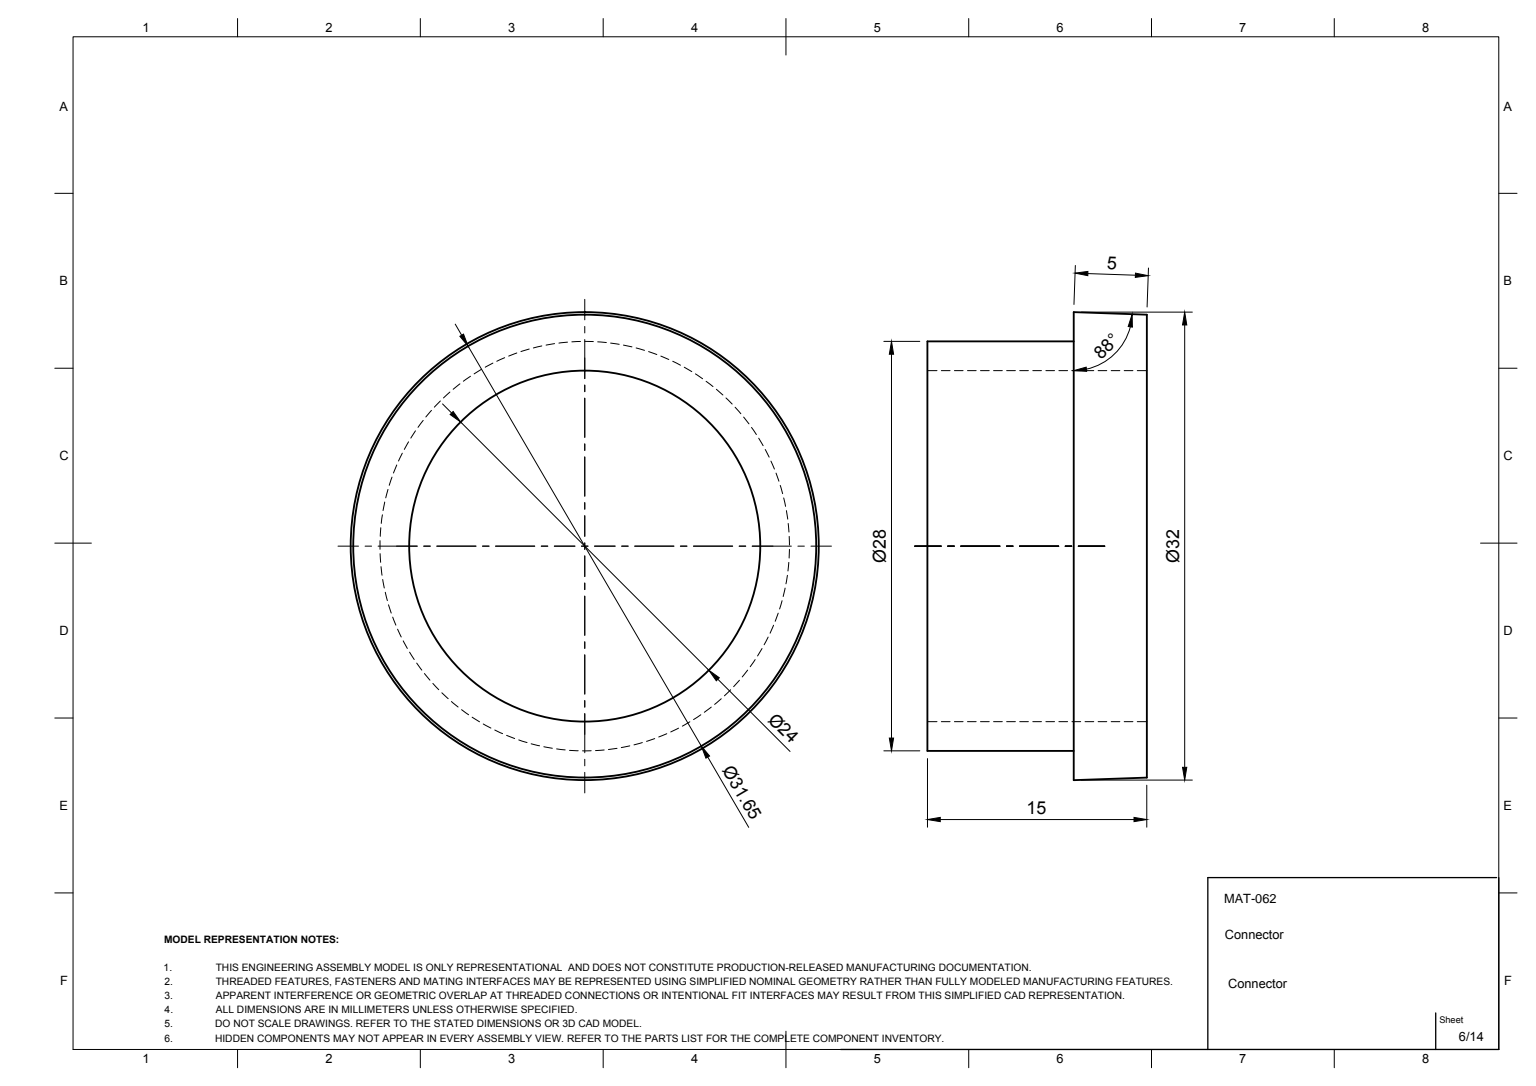
ISO-10303-21;
HEADER;
/* Generated by software containing ST-Developer
 * from STEP Tools, Inc. (www.steptools.com) 
 */

FILE_DESCRIPTION(
/* description */ (''),
/* implementation_level */ '2;1');

FILE_NAME(
/* name */ 'Connector.step',
/* time_stamp */ '2026-10-24T10:18:25-07:00',
/* author */ (''),
/* organization */ (''),
/* preprocessor_version */ 'ST-DEVELOPER v20.2',
/* originating_system */ 'Autodesk Translation Framework v15.15.0.0',
/* authorisation */ '');

FILE_SCHEMA (('AUTOMOTIVE_DESIGN { 1 0 10303 214 3 1 1 }'));
ENDSEC;

DATA;
#10=MECHANICAL_DESIGN_GEOMETRIC_PRESENTATION_REPRESENTATION('',(#265),#14125);
#198=CONICAL_SURFACE('',#6890,16.,0.0349065850398866);
#236=SHAPE_REPRESENTATION_RELATIONSHIP('SRR','None',#14210,#246);
#246=ADVANCED_BREP_SHAPE_REPRESENTATION('',(#278),#14124);
#265=STYLED_ITEM('',(#14263),#278);
#278=MANIFOLD_SOLID_BREP('Connector',#6146);
#625=CYLINDRICAL_SURFACE('',#6897,14.);
#626=CYLINDRICAL_SURFACE('',#6901,12.);
#729=FACE_BOUND('',#1536,.T.);
#730=FACE_BOUND('',#1538,.T.);
#731=FACE_BOUND('',#1541,.T.);
#1079=FACE_OUTER_BOUND('',#1534,.T.);
#1080=FACE_OUTER_BOUND('',#1535,.T.);
#1081=FACE_OUTER_BOUND('',#1537,.T.);
#1082=FACE_OUTER_BOUND('',#1539,.T.);
#1083=FACE_OUTER_BOUND('',#1540,.T.);
#1084=FACE_OUTER_BOUND('',#1542,.T.);
#1534=EDGE_LOOP('',(#5609,#5610,#5611,#5612));
#1535=EDGE_LOOP('',(#5613));
#1536=EDGE_LOOP('',(#5614));
#1537=EDGE_LOOP('',(#5615));
#1538=EDGE_LOOP('',(#5616));
#1539=EDGE_LOOP('',(#5617,#5618,#5619,#5620));
#1540=EDGE_LOOP('',(#5621));
#1541=EDGE_LOOP('',(#5622));
#1542=EDGE_LOOP('',(#5623,#5624,#5625,#5626));
#1797=CIRCLE('',#6891,16.);
#1798=CIRCLE('',#6892,15.8253961525413);
#1799=CIRCLE('',#6894,12.);
#1800=CIRCLE('',#6896,14.);
#1801=CIRCLE('',#6898,14.);
#1802=CIRCLE('',#6900,12.);
#2188=LINE('',#14078,#2576);
#2189=LINE('',#14088,#2577);
#2190=LINE('',#14094,#2578);
#2576=VECTOR('',#8560,16.);
#2577=VECTOR('',#8573,14.);
#2578=VECTOR('',#8582,12.);
#3122=VERTEX_POINT('',#14075);
#3123=VERTEX_POINT('',#14077);
#3124=VERTEX_POINT('',#14081);
#3125=VERTEX_POINT('',#14084);
#3126=VERTEX_POINT('',#14087);
#3127=VERTEX_POINT('',#14091);
#3952=EDGE_CURVE('',#3122,#3122,#1797,.T.);
#3953=EDGE_CURVE('',#3122,#3123,#2188,.T.);
#3954=EDGE_CURVE('',#3123,#3123,#1798,.T.);
#3955=EDGE_CURVE('',#3124,#3124,#1799,.T.);
#3956=EDGE_CURVE('',#3125,#3125,#1800,.T.);
#3957=EDGE_CURVE('',#3125,#3126,#2189,.T.);
#3958=EDGE_CURVE('',#3126,#3126,#1801,.T.);
#3959=EDGE_CURVE('',#3127,#3127,#1802,.T.);
#3960=EDGE_CURVE('',#3124,#3127,#2190,.T.);
#5609=ORIENTED_EDGE('',*,*,#3952,.F.);
#5610=ORIENTED_EDGE('',*,*,#3953,.T.);
#5611=ORIENTED_EDGE('',*,*,#3954,.T.);
#5612=ORIENTED_EDGE('',*,*,#3953,.F.);
#5613=ORIENTED_EDGE('',*,*,#3954,.F.);
#5614=ORIENTED_EDGE('',*,*,#3955,.T.);
#5615=ORIENTED_EDGE('',*,*,#3952,.T.);
#5616=ORIENTED_EDGE('',*,*,#3956,.F.);
#5617=ORIENTED_EDGE('',*,*,#3956,.T.);
#5618=ORIENTED_EDGE('',*,*,#3957,.T.);
#5619=ORIENTED_EDGE('',*,*,#3958,.F.);
#5620=ORIENTED_EDGE('',*,*,#3957,.F.);
#5621=ORIENTED_EDGE('',*,*,#3958,.T.);
#5622=ORIENTED_EDGE('',*,*,#3959,.F.);
#5623=ORIENTED_EDGE('',*,*,#3955,.F.);
#5624=ORIENTED_EDGE('',*,*,#3960,.T.);
#5625=ORIENTED_EDGE('',*,*,#3959,.T.);
#5626=ORIENTED_EDGE('',*,*,#3960,.F.);
#5778=PLANE('',#6893);
#5779=PLANE('',#6895);
#5780=PLANE('',#6899);
#6128=ADVANCED_FACE('',(#1079),#198,.T.);
#6129=ADVANCED_FACE('',(#1080,#729),#5778,.F.);
#6130=ADVANCED_FACE('',(#1081,#730),#5779,.T.);
#6131=ADVANCED_FACE('',(#1082),#625,.T.);
#6132=ADVANCED_FACE('',(#1083,#731),#5780,.T.);
#6133=ADVANCED_FACE('',(#1084),#626,.F.);
#6146=CLOSED_SHELL('',(#6128,#6129,#6130,#6131,#6132,#6133));
#6889=AXIS2_PLACEMENT_3D('',#14073,#8554,#8555);
#6890=AXIS2_PLACEMENT_3D('',#14074,#8556,#8557);
#6891=AXIS2_PLACEMENT_3D('',#14076,#8558,#8559);
#6892=AXIS2_PLACEMENT_3D('',#14079,#8561,#8562);
#6893=AXIS2_PLACEMENT_3D('',#14080,#8563,#8564);
#6894=AXIS2_PLACEMENT_3D('',#14082,#8565,#8566);
#6895=AXIS2_PLACEMENT_3D('',#14083,#8567,#8568);
#6896=AXIS2_PLACEMENT_3D('',#14085,#8569,#8570);
#6897=AXIS2_PLACEMENT_3D('',#14086,#8571,#8572);
#6898=AXIS2_PLACEMENT_3D('',#14089,#8574,#8575);
#6899=AXIS2_PLACEMENT_3D('',#14090,#8576,#8577);
#6900=AXIS2_PLACEMENT_3D('',#14092,#8578,#8579);
#6901=AXIS2_PLACEMENT_3D('',#14093,#8580,#8581);
#8554=DIRECTION('axis',(0.,0.,1.));
#8555=DIRECTION('refdir',(1.,0.,0.));
#8556=DIRECTION('center_axis',(0.,-1.,0.));
#8557=DIRECTION('ref_axis',(0.,0.,-1.));
#8558=DIRECTION('center_axis',(0.,-1.,0.));
#8559=DIRECTION('ref_axis',(0.,0.,-1.));
#8560=DIRECTION('',(4.27395569285715E-18,0.999390827019096,-0.034899496702501));
#8561=DIRECTION('center_axis',(0.,-1.,0.));
#8562=DIRECTION('ref_axis',(0.,0.,-1.));
#8563=DIRECTION('center_axis',(0.,-1.,0.));
#8564=DIRECTION('ref_axis',(0.,0.,-1.));
#8565=DIRECTION('center_axis',(0.,-1.,0.));
#8566=DIRECTION('ref_axis',(0.,0.,-1.));
#8567=DIRECTION('center_axis',(0.,-1.,0.));
#8568=DIRECTION('ref_axis',(0.,0.,-1.));
#8569=DIRECTION('center_axis',(0.,-1.,0.));
#8570=DIRECTION('ref_axis',(0.,0.,-1.));
#8571=DIRECTION('center_axis',(0.,1.,0.));
#8572=DIRECTION('ref_axis',(0.,0.,1.));
#8573=DIRECTION('',(0.,-1.,0.));
#8574=DIRECTION('center_axis',(0.,-1.,0.));
#8575=DIRECTION('ref_axis',(0.,0.,-1.));
#8576=DIRECTION('center_axis',(0.,-1.,0.));
#8577=DIRECTION('ref_axis',(0.,0.,-1.));
#8578=DIRECTION('center_axis',(0.,-1.,0.));
#8579=DIRECTION('ref_axis',(0.,0.,-1.));
#8580=DIRECTION('center_axis',(0.,-1.,0.));
#8581=DIRECTION('ref_axis',(0.,0.,-1.));
#8582=DIRECTION('',(0.,-1.,0.));
#14073=CARTESIAN_POINT('',(0.,0.,0.));
#14074=CARTESIAN_POINT('Origin',(0.,89.,-11.9999999999999));
#14075=CARTESIAN_POINT('',(-1.95943487863577E-15,89.,4.00000000000008));
#14076=CARTESIAN_POINT('Origin',(0.,89.,-11.9999999999999));
#14077=CARTESIAN_POINT('',(-1.93805207434485E-15,94.,3.82539615254134));
#14078=CARTESIAN_POINT('',(-1.95943487863577E-15,89.,4.00000000000008));
#14079=CARTESIAN_POINT('Origin',(0.,94.,-11.9999999999999));
#14080=CARTESIAN_POINT('Origin',(0.,94.,-11.9999999999999));
#14081=CARTESIAN_POINT('',(-1.46957615897682E-15,94.,8.21565038222616E-14));
#14082=CARTESIAN_POINT('Origin',(0.,94.,-11.9999999999999));
#14083=CARTESIAN_POINT('Origin',(0.,89.,-11.9999999999999));
#14084=CARTESIAN_POINT('',(0.,89.,-25.9999999999999));
#14085=CARTESIAN_POINT('Origin',(0.,89.,-11.9999999999999));
#14086=CARTESIAN_POINT('Origin',(0.,79.,-11.9999999999999));
#14087=CARTESIAN_POINT('',(0.,79.,-25.9999999999999));
#14088=CARTESIAN_POINT('',(-1.71450551880629E-15,79.,-25.9999999999999));
#14089=CARTESIAN_POINT('Origin',(0.,79.,-11.9999999999999));
#14090=CARTESIAN_POINT('Origin',(0.,79.,-11.9999999999999));
#14091=CARTESIAN_POINT('',(-1.46957615897682E-15,79.,8.21565038222616E-14));
#14092=CARTESIAN_POINT('Origin',(0.,79.,-11.9999999999999));
#14093=CARTESIAN_POINT('Origin',(0.,136.,-11.9999999999999));
#14094=CARTESIAN_POINT('',(-1.46957615897682E-15,136.,8.21565038222616E-14));
#14111=UNCERTAINTY_MEASURE_WITH_UNIT(LENGTH_MEASURE(0.01),#14126,
'DISTANCE_ACCURACY_VALUE',
'Maximum model space distance between geometric entities at asserted c
onnectivities');
#14112=UNCERTAINTY_MEASURE_WITH_UNIT(LENGTH_MEASURE(0.01),#14126,
'DISTANCE_ACCURACY_VALUE',
'Maximum model space distance between geometric entities at asserted c
onnectivities');
#14124=(
GEOMETRIC_REPRESENTATION_CONTEXT(3)
GLOBAL_UNCERTAINTY_ASSIGNED_CONTEXT((#14111))
GLOBAL_UNIT_ASSIGNED_CONTEXT((#14126,#14128,#14129))
REPRESENTATION_CONTEXT('','3D')
);
#14125=(
GEOMETRIC_REPRESENTATION_CONTEXT(3)
GLOBAL_UNCERTAINTY_ASSIGNED_CONTEXT((#14112))
GLOBAL_UNIT_ASSIGNED_CONTEXT((#14126,#14128,#14129))
REPRESENTATION_CONTEXT('','3D')
);
#14126=(
LENGTH_UNIT()
NAMED_UNIT(*)
SI_UNIT(.MILLI.,.METRE.)
);
#14128=(
NAMED_UNIT(*)
PLANE_ANGLE_UNIT()
SI_UNIT($,.RADIAN.)
);
#14129=(
NAMED_UNIT(*)
SI_UNIT($,.STERADIAN.)
SOLID_ANGLE_UNIT()
);
#14141=SHAPE_DEFINITION_REPRESENTATION(#14193,#14210);
#14193=PRODUCT_DEFINITION_SHAPE('',$,#14223);
#14210=SHAPE_REPRESENTATION('',(#6889),#14124);
#14211=PRODUCT_DEFINITION_CONTEXT('part definition',#14249,'design');
#14223=PRODUCT_DEFINITION('Connector','Connector',#14235,#14211);
#14235=PRODUCT_DEFINITION_FORMATION('',$,#14262);
#14249=APPLICATION_CONTEXT(
'Core Data for Automotive Mechanical Design Process');
#14250=PRODUCT_CONTEXT('part definition',#14249,'mechanical');
#14262=PRODUCT('Connector','Connector',$,(#14250));
#14263=PRESENTATION_STYLE_ASSIGNMENT((#14265));
#14265=SURFACE_STYLE_USAGE(.BOTH.,#14267);
#14267=SURFACE_SIDE_STYLE('',(#14269));
#14269=SURFACE_STYLE_FILL_AREA(#14271);
#14271=FILL_AREA_STYLE('Steel - Satin',(#14273));
#14273=FILL_AREA_STYLE_COLOUR('Steel - Satin',#14275);
#14275=COLOUR_RGB('Steel - Satin',0.627450980392157,0.627450980392157,0.627450980392157);
ENDSEC;
END-ISO-10303-21;
